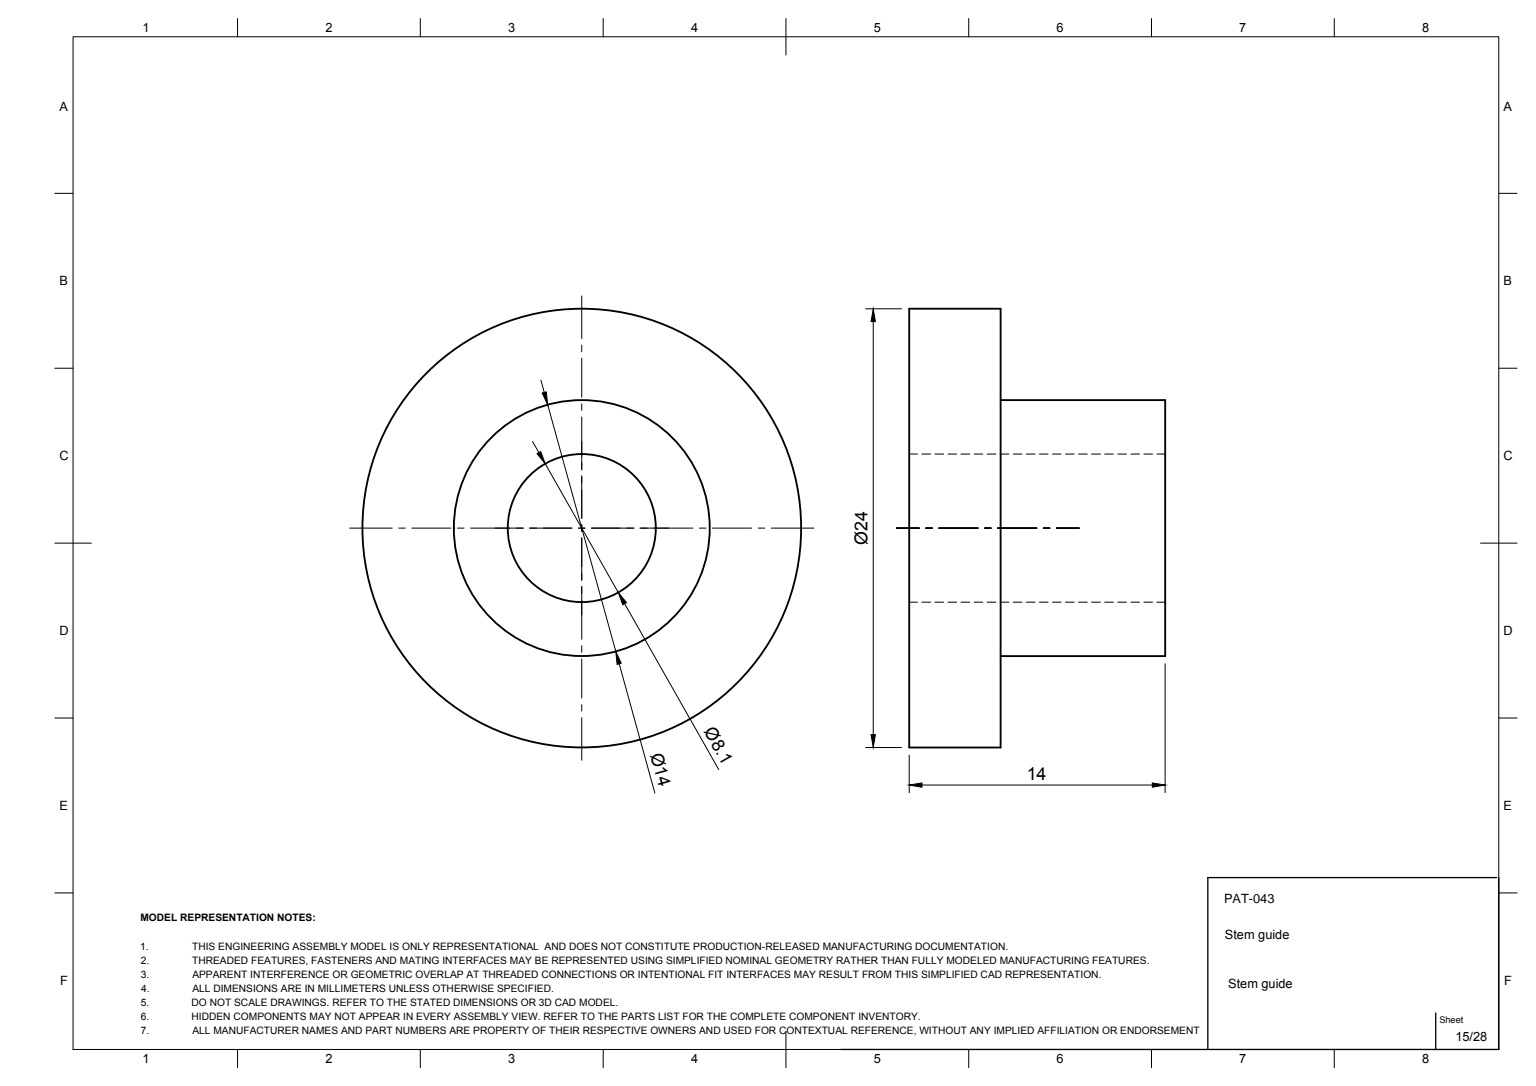
ISO-10303-21;
HEADER;
/* Generated by software containing ST-Developer
 * from STEP Tools, Inc. (www.steptools.com) 
 */

FILE_DESCRIPTION(
/* description */ ('Four-valve pipe header'),
/* implementation_level */ '2;1');

FILE_NAME(
/* name */ 'Stem guide.step',
/* time_stamp */ '2026-10-29T16:56:19-07:00',
/* author */ (''),
/* organization */ (''),
/* preprocessor_version */ 'ST-DEVELOPER v20.2',
/* originating_system */ 'Autodesk Translation Framework v15.17.0.0',
/* authorisation */ '');

FILE_SCHEMA (('AUTOMOTIVE_DESIGN { 1 0 10303 214 3 1 1 }'));
ENDSEC;

DATA;
#10=MECHANICAL_DESIGN_GEOMETRIC_PRESENTATION_REPRESENTATION('',(#341),#10119);
#289=SHAPE_REPRESENTATION_RELATIONSHIP('SRR','None',#10251,#315);
#315=ADVANCED_BREP_SHAPE_REPRESENTATION('',(#367),#10100);
#341=STYLED_ITEM('',(#10463),#367);
#367=MANIFOLD_SOLID_BREP('Body1',#5587);
#492=FACE_BOUND('',#1307,.T.);
#493=FACE_BOUND('',#1310,.T.);
#494=FACE_BOUND('',#1314,.T.);
#630=PLANE('',#6220);
#631=PLANE('',#6225);
#632=PLANE('',#6231);
#908=FACE_OUTER_BOUND('',#1306,.T.);
#909=FACE_OUTER_BOUND('',#1308,.T.);
#910=FACE_OUTER_BOUND('',#1309,.T.);
#911=FACE_OUTER_BOUND('',#1311,.T.);
#912=FACE_OUTER_BOUND('',#1312,.T.);
#913=FACE_OUTER_BOUND('',#1313,.T.);
#1306=EDGE_LOOP('',(#4483));
#1307=EDGE_LOOP('',(#4484));
#1308=EDGE_LOOP('',(#4485,#4486,#4487,#4488));
#1309=EDGE_LOOP('',(#4489));
#1310=EDGE_LOOP('',(#4490));
#1311=EDGE_LOOP('',(#4491,#4492,#4493,#4494));
#1312=EDGE_LOOP('',(#4495,#4496,#4497,#4498));
#1313=EDGE_LOOP('',(#4499));
#1314=EDGE_LOOP('',(#4500));
#1721=LINE('',#9249,#2139);
#1722=LINE('',#9255,#2140);
#1723=LINE('',#9259,#2141);
#2139=VECTOR('',#7430,1.2);
#2140=VECTOR('',#7437,0.405);
#2141=VECTOR('',#7442,0.7);
#2476=CIRCLE('',#6221,1.2);
#2477=CIRCLE('',#6222,0.7);
#2478=CIRCLE('',#6224,1.2);
#2479=CIRCLE('',#6226,0.405);
#2480=CIRCLE('',#6228,0.405);
#2481=CIRCLE('',#6230,0.7);
#2822=VERTEX_POINT('',#9242);
#2823=VERTEX_POINT('',#9244);
#2824=VERTEX_POINT('',#9247);
#2825=VERTEX_POINT('',#9251);
#2826=VERTEX_POINT('',#9254);
#2827=VERTEX_POINT('',#9258);
#3408=EDGE_CURVE('',#2822,#2822,#2476,.T.);
#3409=EDGE_CURVE('',#2823,#2823,#2477,.T.);
#3410=EDGE_CURVE('',#2824,#2824,#2478,.T.);
#3411=EDGE_CURVE('',#2824,#2822,#1721,.T.);
#3412=EDGE_CURVE('',#2825,#2825,#2479,.T.);
#3413=EDGE_CURVE('',#2825,#2826,#1722,.T.);
#3414=EDGE_CURVE('',#2826,#2826,#2480,.T.);
#3415=EDGE_CURVE('',#2823,#2827,#1723,.T.);
#3416=EDGE_CURVE('',#2827,#2827,#2481,.T.);
#4483=ORIENTED_EDGE('',*,*,#3408,.F.);
#4484=ORIENTED_EDGE('',*,*,#3409,.T.);
#4485=ORIENTED_EDGE('',*,*,#3410,.F.);
#4486=ORIENTED_EDGE('',*,*,#3411,.T.);
#4487=ORIENTED_EDGE('',*,*,#3408,.T.);
#4488=ORIENTED_EDGE('',*,*,#3411,.F.);
#4489=ORIENTED_EDGE('',*,*,#3410,.T.);
#4490=ORIENTED_EDGE('',*,*,#3412,.T.);
#4491=ORIENTED_EDGE('',*,*,#3412,.F.);
#4492=ORIENTED_EDGE('',*,*,#3413,.T.);
#4493=ORIENTED_EDGE('',*,*,#3414,.T.);
#4494=ORIENTED_EDGE('',*,*,#3413,.F.);
#4495=ORIENTED_EDGE('',*,*,#3409,.F.);
#4496=ORIENTED_EDGE('',*,*,#3415,.T.);
#4497=ORIENTED_EDGE('',*,*,#3416,.T.);
#4498=ORIENTED_EDGE('',*,*,#3415,.F.);
#4499=ORIENTED_EDGE('',*,*,#3416,.F.);
#4500=ORIENTED_EDGE('',*,*,#3414,.F.);
#5211=CYLINDRICAL_SURFACE('',#6223,1.2);
#5212=CYLINDRICAL_SURFACE('',#6227,0.405);
#5213=CYLINDRICAL_SURFACE('',#6229,0.7);
#5408=ADVANCED_FACE('',(#908,#492),#630,.F.);
#5409=ADVANCED_FACE('',(#909),#5211,.T.);
#5410=ADVANCED_FACE('',(#910,#493),#631,.T.);
#5411=ADVANCED_FACE('',(#911),#5212,.F.);
#5412=ADVANCED_FACE('',(#912),#5213,.T.);
#5413=ADVANCED_FACE('',(#913,#494),#632,.F.);
#5587=CLOSED_SHELL('',(#5408,#5409,#5410,#5411,#5412,#5413));
#6219=AXIS2_PLACEMENT_3D('',#9240,#7418,#7419);
#6220=AXIS2_PLACEMENT_3D('',#9241,#7420,#7421);
#6221=AXIS2_PLACEMENT_3D('',#9243,#7422,#7423);
#6222=AXIS2_PLACEMENT_3D('',#9245,#7424,#7425);
#6223=AXIS2_PLACEMENT_3D('',#9246,#7426,#7427);
#6224=AXIS2_PLACEMENT_3D('',#9248,#7428,#7429);
#6225=AXIS2_PLACEMENT_3D('',#9250,#7431,#7432);
#6226=AXIS2_PLACEMENT_3D('',#9252,#7433,#7434);
#6227=AXIS2_PLACEMENT_3D('',#9253,#7435,#7436);
#6228=AXIS2_PLACEMENT_3D('',#9256,#7438,#7439);
#6229=AXIS2_PLACEMENT_3D('',#9257,#7440,#7441);
#6230=AXIS2_PLACEMENT_3D('',#9260,#7443,#7444);
#6231=AXIS2_PLACEMENT_3D('',#9261,#7445,#7446);
#7418=DIRECTION('axis',(0.,0.,1.));
#7419=DIRECTION('refdir',(1.,0.,0.));
#7420=DIRECTION('center_axis',(0.,0.,1.));
#7421=DIRECTION('ref_axis',(1.,0.,0.));
#7422=DIRECTION('center_axis',(0.,0.,1.));
#7423=DIRECTION('ref_axis',(1.,0.,0.));
#7424=DIRECTION('center_axis',(0.,0.,1.));
#7425=DIRECTION('ref_axis',(1.,0.,0.));
#7426=DIRECTION('center_axis',(0.,0.,1.));
#7427=DIRECTION('ref_axis',(1.,0.,0.));
#7428=DIRECTION('center_axis',(0.,0.,1.));
#7429=DIRECTION('ref_axis',(1.,0.,0.));
#7430=DIRECTION('',(0.,0.,-1.));
#7431=DIRECTION('center_axis',(0.,0.,1.));
#7432=DIRECTION('ref_axis',(1.,0.,0.));
#7433=DIRECTION('center_axis',(0.,0.,-1.));
#7434=DIRECTION('ref_axis',(1.,0.,0.));
#7435=DIRECTION('center_axis',(0.,0.,1.));
#7436=DIRECTION('ref_axis',(1.,0.,0.));
#7437=DIRECTION('',(0.,0.,-1.));
#7438=DIRECTION('center_axis',(0.,0.,-1.));
#7439=DIRECTION('ref_axis',(1.,0.,0.));
#7440=DIRECTION('center_axis',(0.,0.,1.));
#7441=DIRECTION('ref_axis',(1.,0.,0.));
#7442=DIRECTION('',(0.,0.,-1.));
#7443=DIRECTION('center_axis',(0.,0.,1.));
#7444=DIRECTION('ref_axis',(1.,0.,0.));
#7445=DIRECTION('center_axis',(0.,0.,1.));
#7446=DIRECTION('ref_axis',(1.,0.,0.));
#9240=CARTESIAN_POINT('',(0.,0.,0.));
#9241=CARTESIAN_POINT('Origin',(0.,0.,7.5));
#9242=CARTESIAN_POINT('',(-1.2,-1.46957615897682E-16,7.5));
#9243=CARTESIAN_POINT('Origin',(0.,0.,7.5));
#9244=CARTESIAN_POINT('',(-0.7,-8.57252759403147E-17,7.5));
#9245=CARTESIAN_POINT('Origin',(0.,0.,7.5));
#9246=CARTESIAN_POINT('Origin',(0.,0.,7.5));
#9247=CARTESIAN_POINT('',(-1.2,-1.46957615897682E-16,8.));
#9248=CARTESIAN_POINT('Origin',(0.,0.,8.));
#9249=CARTESIAN_POINT('',(-1.2,-1.46957615897682E-16,7.5));
#9250=CARTESIAN_POINT('Origin',(0.,0.,8.));
#9251=CARTESIAN_POINT('',(-0.405,-4.95981953654678E-17,8.));
#9252=CARTESIAN_POINT('Origin',(0.,0.,8.));
#9253=CARTESIAN_POINT('Origin',(0.,0.,6.6));
#9254=CARTESIAN_POINT('',(-0.405,-4.95981953654678E-17,6.6));
#9255=CARTESIAN_POINT('',(-0.405,-4.95981953654678E-17,6.6));
#9256=CARTESIAN_POINT('Origin',(0.,0.,6.6));
#9257=CARTESIAN_POINT('Origin',(0.,0.,6.6));
#9258=CARTESIAN_POINT('',(-0.7,-8.57252759403147E-17,6.6));
#9259=CARTESIAN_POINT('',(-0.7,-8.57252759403147E-17,6.6));
#9260=CARTESIAN_POINT('Origin',(0.,0.,6.6));
#9261=CARTESIAN_POINT('Origin',(0.,0.,6.6));
#10069=UNCERTAINTY_MEASURE_WITH_UNIT(LENGTH_MEASURE(0.001),#10120,
'DISTANCE_ACCURACY_VALUE',
'Maximum model space distance between geometric entities at asserted c
onnectivities');
#10088=UNCERTAINTY_MEASURE_WITH_UNIT(LENGTH_MEASURE(0.001),#10120,
'DISTANCE_ACCURACY_VALUE',
'Maximum model space distance between geometric entities at asserted c
onnectivities');
#10100=(
GEOMETRIC_REPRESENTATION_CONTEXT(3)
GLOBAL_UNCERTAINTY_ASSIGNED_CONTEXT((#10069))
GLOBAL_UNIT_ASSIGNED_CONTEXT((#10120,#10122,#10123))
REPRESENTATION_CONTEXT('','3D')
);
#10119=(
GEOMETRIC_REPRESENTATION_CONTEXT(3)
GLOBAL_UNCERTAINTY_ASSIGNED_CONTEXT((#10088))
GLOBAL_UNIT_ASSIGNED_CONTEXT((#10120,#10122,#10123))
REPRESENTATION_CONTEXT('','3D')
);
#10120=(
LENGTH_UNIT()
NAMED_UNIT(*)
SI_UNIT(.CENTI.,.METRE.)
);
#10122=(
NAMED_UNIT(*)
PLANE_ANGLE_UNIT()
SI_UNIT($,.RADIAN.)
);
#10123=(
NAMED_UNIT(*)
SI_UNIT($,.STERADIAN.)
SOLID_ANGLE_UNIT()
);
#10135=SHAPE_DEFINITION_REPRESENTATION(#10165,#10251);
#10165=PRODUCT_DEFINITION_SHAPE('',$,#10282);
#10251=SHAPE_REPRESENTATION('',(#6219),#10100);
#10270=PRODUCT_DEFINITION_CONTEXT('part definition',#10362,'design');
#10282=PRODUCT_DEFINITION('Stem guide','Stem guide',#10312,#10270);
#10312=PRODUCT_DEFINITION_FORMATION('',$,#10375);
#10362=APPLICATION_CONTEXT(
'Core Data for Automotive Mechanical Design Process');
#10363=PRODUCT_CONTEXT('part definition',#10362,'mechanical');
#10375=PRODUCT('Stem guide','Stem guide','Stem guide',(#10363));
#10457=COLOUR_RGB('Sky Blue',0.24,0.69,0.87);
#10458=FILL_AREA_STYLE_COLOUR('',#10457);
#10459=FILL_AREA_STYLE('',(#10458));
#10460=SURFACE_STYLE_FILL_AREA(#10459);
#10461=SURFACE_SIDE_STYLE('',(#10460));
#10462=SURFACE_STYLE_USAGE(.BOTH.,#10461);
#10463=PRESENTATION_STYLE_ASSIGNMENT((#10462));
ENDSEC;
END-ISO-10303-21;
